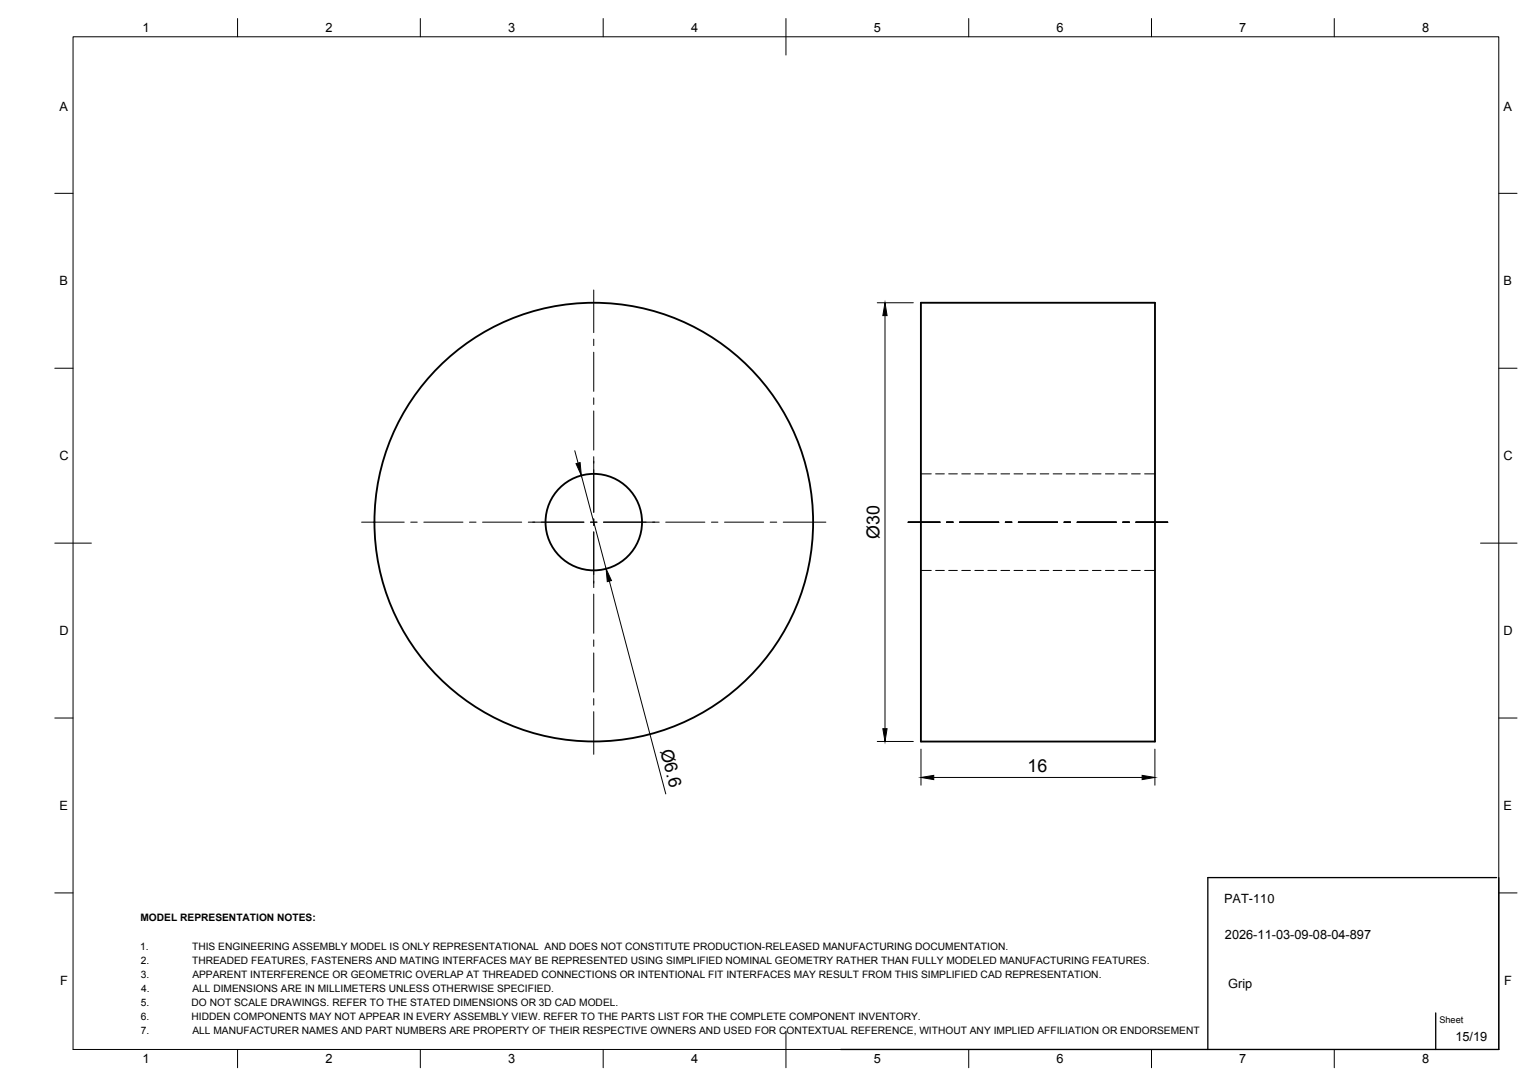
ISO-10303-21;
HEADER;
/* Generated by software containing ST-Developer
 * from STEP Tools, Inc. (www.steptools.com) 
 */

FILE_DESCRIPTION(
/* description */ ('Twin-shaft manual slide'),
/* implementation_level */ '2;1');

FILE_NAME(
/* name */ 'Grip.step',
/* time_stamp */ '2026-10-27T18:38:08-07:00',
/* author */ (''),
/* organization */ (''),
/* preprocessor_version */ 'ST-DEVELOPER v20.2',
/* originating_system */ 'Autodesk Translation Framework v15.17.0.0',
/* authorisation */ '');

FILE_SCHEMA (('AUTOMOTIVE_DESIGN { 1 0 10303 214 3 1 1 }'));
ENDSEC;

DATA;
#10=MECHANICAL_DESIGN_GEOMETRIC_PRESENTATION_REPRESENTATION('',(#289),#6463);
#257=SHAPE_REPRESENTATION_RELATIONSHIP('SRR','None',#6577,#273);
#273=ADVANCED_BREP_SHAPE_REPRESENTATION('',(#302),#6460);
#289=STYLED_ITEM('',(#6747),#302);
#302=MANIFOLD_SOLID_BREP('Body1',#3654);
#396=FACE_BOUND('',#1010,.T.);
#397=FACE_BOUND('',#1012,.T.);
#511=PLANE('',#4207);
#512=PLANE('',#4208);
#708=FACE_OUTER_BOUND('',#1007,.T.);
#709=FACE_OUTER_BOUND('',#1008,.T.);
#710=FACE_OUTER_BOUND('',#1009,.T.);
#711=FACE_OUTER_BOUND('',#1011,.T.);
#1007=EDGE_LOOP('',(#3278,#3279,#3280,#3281));
#1008=EDGE_LOOP('',(#3282,#3283,#3284,#3285));
#1009=EDGE_LOOP('',(#3286));
#1010=EDGE_LOOP('',(#3287));
#1011=EDGE_LOOP('',(#3288));
#1012=EDGE_LOOP('',(#3289));
#1295=LINE('',#6304,#1581);
#1296=LINE('',#6310,#1582);
#1581=VECTOR('',#5261,0.33);
#1582=VECTOR('',#5268,1.5);
#1746=CIRCLE('',#4202,0.33);
#1747=CIRCLE('',#4203,0.33);
#1748=CIRCLE('',#4205,1.5);
#1749=CIRCLE('',#4206,1.5);
#2021=VERTEX_POINT('',#6301);
#2022=VERTEX_POINT('',#6303);
#2023=VERTEX_POINT('',#6307);
#2024=VERTEX_POINT('',#6309);
#2444=EDGE_CURVE('',#2021,#2021,#1746,.T.);
#2445=EDGE_CURVE('',#2021,#2022,#1295,.T.);
#2446=EDGE_CURVE('',#2022,#2022,#1747,.T.);
#2447=EDGE_CURVE('',#2023,#2023,#1748,.T.);
#2448=EDGE_CURVE('',#2023,#2024,#1296,.T.);
#2449=EDGE_CURVE('',#2024,#2024,#1749,.T.);
#3278=ORIENTED_EDGE('',*,*,#2444,.F.);
#3279=ORIENTED_EDGE('',*,*,#2445,.T.);
#3280=ORIENTED_EDGE('',*,*,#2446,.T.);
#3281=ORIENTED_EDGE('',*,*,#2445,.F.);
#3282=ORIENTED_EDGE('',*,*,#2447,.F.);
#3283=ORIENTED_EDGE('',*,*,#2448,.T.);
#3284=ORIENTED_EDGE('',*,*,#2449,.T.);
#3285=ORIENTED_EDGE('',*,*,#2448,.F.);
#3286=ORIENTED_EDGE('',*,*,#2447,.T.);
#3287=ORIENTED_EDGE('',*,*,#2444,.T.);
#3288=ORIENTED_EDGE('',*,*,#2449,.F.);
#3289=ORIENTED_EDGE('',*,*,#2446,.F.);
#3425=CYLINDRICAL_SURFACE('',#4201,0.33);
#3426=CYLINDRICAL_SURFACE('',#4204,1.5);
#3613=ADVANCED_FACE('',(#708),#3425,.F.);
#3614=ADVANCED_FACE('',(#709),#3426,.T.);
#3615=ADVANCED_FACE('',(#710,#396),#511,.T.);
#3616=ADVANCED_FACE('',(#711,#397),#512,.F.);
#3654=CLOSED_SHELL('',(#3613,#3614,#3615,#3616));
#4200=AXIS2_PLACEMENT_3D('',#6299,#5255,#5256);
#4201=AXIS2_PLACEMENT_3D('',#6300,#5257,#5258);
#4202=AXIS2_PLACEMENT_3D('',#6302,#5259,#5260);
#4203=AXIS2_PLACEMENT_3D('',#6305,#5262,#5263);
#4204=AXIS2_PLACEMENT_3D('',#6306,#5264,#5265);
#4205=AXIS2_PLACEMENT_3D('',#6308,#5266,#5267);
#4206=AXIS2_PLACEMENT_3D('',#6311,#5269,#5270);
#4207=AXIS2_PLACEMENT_3D('',#6312,#5271,#5272);
#4208=AXIS2_PLACEMENT_3D('',#6313,#5273,#5274);
#5255=DIRECTION('axis',(0.,0.,1.));
#5256=DIRECTION('refdir',(1.,0.,0.));
#5257=DIRECTION('center_axis',(0.,0.,1.));
#5258=DIRECTION('ref_axis',(1.,0.,0.));
#5259=DIRECTION('center_axis',(0.,0.,-1.));
#5260=DIRECTION('ref_axis',(1.,0.,0.));
#5261=DIRECTION('',(0.,0.,-1.));
#5262=DIRECTION('center_axis',(0.,0.,-1.));
#5263=DIRECTION('ref_axis',(1.,0.,0.));
#5264=DIRECTION('center_axis',(0.,0.,1.));
#5265=DIRECTION('ref_axis',(1.,0.,0.));
#5266=DIRECTION('center_axis',(0.,0.,1.));
#5267=DIRECTION('ref_axis',(1.,0.,0.));
#5268=DIRECTION('',(0.,0.,-1.));
#5269=DIRECTION('center_axis',(0.,0.,1.));
#5270=DIRECTION('ref_axis',(1.,0.,0.));
#5271=DIRECTION('center_axis',(0.,0.,1.));
#5272=DIRECTION('ref_axis',(1.,0.,0.));
#5273=DIRECTION('center_axis',(0.,0.,1.));
#5274=DIRECTION('ref_axis',(1.,0.,0.));
#6299=CARTESIAN_POINT('',(0.,0.,0.));
#6300=CARTESIAN_POINT('Origin',(15.,0.,6.6));
#6301=CARTESIAN_POINT('',(14.67,-4.04133443718627E-17,8.2));
#6302=CARTESIAN_POINT('Origin',(15.,0.,8.2));
#6303=CARTESIAN_POINT('',(14.67,-4.04133443718627E-17,6.6));
#6304=CARTESIAN_POINT('',(14.67,-4.04133443718627E-17,6.6));
#6305=CARTESIAN_POINT('Origin',(15.,0.,6.6));
#6306=CARTESIAN_POINT('Origin',(15.,0.,6.6));
#6307=CARTESIAN_POINT('',(13.5,-1.83697019872103E-16,8.2));
#6308=CARTESIAN_POINT('Origin',(15.,0.,8.2));
#6309=CARTESIAN_POINT('',(13.5,-1.83697019872103E-16,6.6));
#6310=CARTESIAN_POINT('',(13.5,-1.83697019872103E-16,6.6));
#6311=CARTESIAN_POINT('Origin',(15.,0.,6.6));
#6312=CARTESIAN_POINT('Origin',(15.,0.,8.2));
#6313=CARTESIAN_POINT('Origin',(15.,0.,6.6));
#6439=UNCERTAINTY_MEASURE_WITH_UNIT(LENGTH_MEASURE(0.001),#6464,
'DISTANCE_ACCURACY_VALUE',
'Maximum model space distance between geometric entities at asserted c
onnectivities');
#6442=UNCERTAINTY_MEASURE_WITH_UNIT(LENGTH_MEASURE(0.001),#6464,
'DISTANCE_ACCURACY_VALUE',
'Maximum model space distance between geometric entities at asserted c
onnectivities');
#6460=(
GEOMETRIC_REPRESENTATION_CONTEXT(3)
GLOBAL_UNCERTAINTY_ASSIGNED_CONTEXT((#6439))
GLOBAL_UNIT_ASSIGNED_CONTEXT((#6464,#6466,#6467))
REPRESENTATION_CONTEXT('','3D')
);
#6463=(
GEOMETRIC_REPRESENTATION_CONTEXT(3)
GLOBAL_UNCERTAINTY_ASSIGNED_CONTEXT((#6442))
GLOBAL_UNIT_ASSIGNED_CONTEXT((#6464,#6466,#6467))
REPRESENTATION_CONTEXT('','3D')
);
#6464=(
LENGTH_UNIT()
NAMED_UNIT(*)
SI_UNIT(.CENTI.,.METRE.)
);
#6466=(
NAMED_UNIT(*)
PLANE_ANGLE_UNIT()
SI_UNIT($,.RADIAN.)
);
#6467=(
NAMED_UNIT(*)
SI_UNIT($,.STERADIAN.)
SOLID_ANGLE_UNIT()
);
#6485=SHAPE_DEFINITION_REPRESENTATION(#6534,#6577);
#6534=PRODUCT_DEFINITION_SHAPE('',$,#6598);
#6577=SHAPE_REPRESENTATION('',(#4200),#6460);
#6580=PRODUCT_DEFINITION_CONTEXT('part definition',#6642,'design');
#6598=PRODUCT_DEFINITION('Grip','Grip',#6618,#6580);
#6618=PRODUCT_DEFINITION_FORMATION('',$,#6661);
#6642=APPLICATION_CONTEXT(
'Core Data for Automotive Mechanical Design Process');
#6643=PRODUCT_CONTEXT('part definition',#6642,'mechanical');
#6661=PRODUCT('Grip','Grip','Grip',(#6643));
#6741=COLOUR_RGB('Black',0.12,0.14,0.17);
#6742=FILL_AREA_STYLE_COLOUR('',#6741);
#6743=FILL_AREA_STYLE('',(#6742));
#6744=SURFACE_STYLE_FILL_AREA(#6743);
#6745=SURFACE_SIDE_STYLE('',(#6744));
#6746=SURFACE_STYLE_USAGE(.BOTH.,#6745);
#6747=PRESENTATION_STYLE_ASSIGNMENT((#6746));
ENDSEC;
END-ISO-10303-21;
